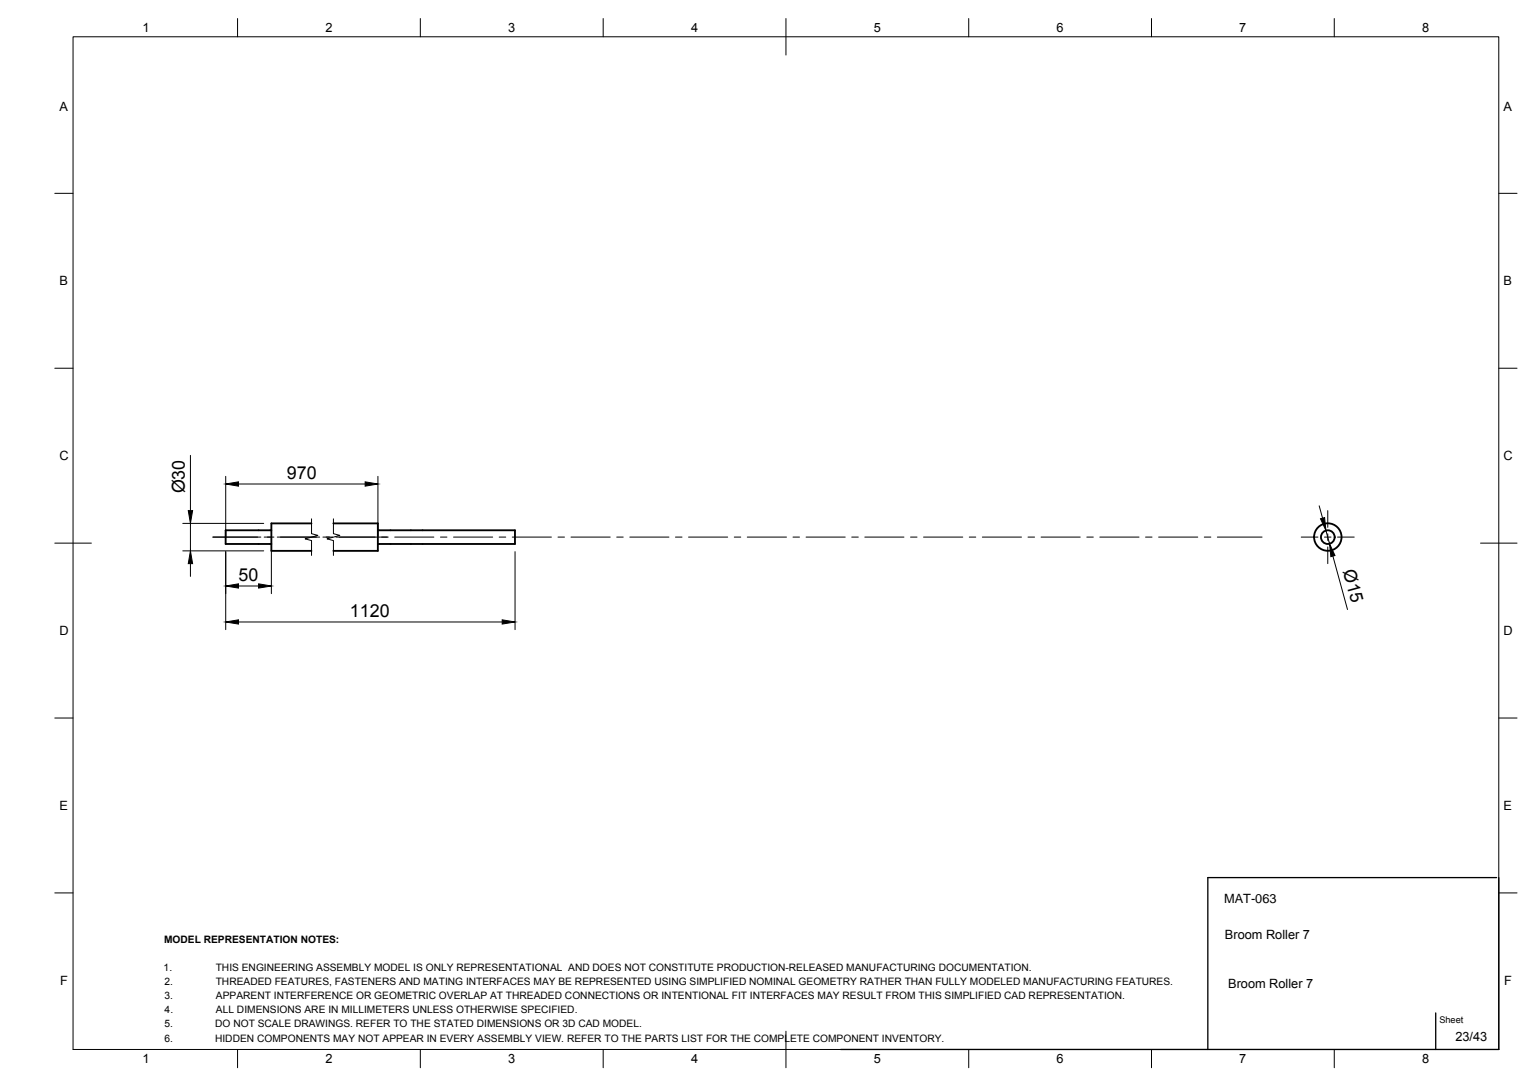
ISO-10303-21;
HEADER;
/* Generated by software containing ST-Developer
 * from STEP Tools, Inc. (www.steptools.com) 
 */

FILE_DESCRIPTION(
/* description */ (''),
/* implementation_level */ '2;1');

FILE_NAME(
/* name */ 'Broom Roller 7.step',
/* time_stamp */ '2026-10-24T09:43:01-07:00',
/* author */ (''),
/* organization */ (''),
/* preprocessor_version */ 'ST-DEVELOPER v20.2',
/* originating_system */ 'Autodesk Translation Framework v15.15.0.0',
/* authorisation */ '');

FILE_SCHEMA (('AUTOMOTIVE_DESIGN { 1 0 10303 214 3 1 1 }'));
ENDSEC;

DATA;
#10=MECHANICAL_DESIGN_GEOMETRIC_PRESENTATION_REPRESENTATION('',(#288),#11112);
#222=SHAPE_REPRESENTATION_RELATIONSHIP('SRR','None',#11246,#255);
#255=ADVANCED_BREP_SHAPE_REPRESENTATION('',(#321),#11091);
#288=STYLED_ITEM('',(#11426),#321);
#321=MANIFOLD_SOLID_BREP('Broom Roller 7',#6025);
#415=FACE_BOUND('',#1337,.T.);
#416=FACE_BOUND('',#1342,.T.);
#588=PLANE('',#6944);
#589=PLANE('',#6950);
#590=PLANE('',#6952);
#591=PLANE('',#6953);
#891=FACE_OUTER_BOUND('',#1331,.T.);
#892=FACE_OUTER_BOUND('',#1332,.T.);
#893=FACE_OUTER_BOUND('',#1333,.T.);
#894=FACE_OUTER_BOUND('',#1334,.T.);
#895=FACE_OUTER_BOUND('',#1335,.T.);
#896=FACE_OUTER_BOUND('',#1336,.T.);
#897=FACE_OUTER_BOUND('',#1338,.T.);
#898=FACE_OUTER_BOUND('',#1339,.T.);
#899=FACE_OUTER_BOUND('',#1340,.T.);
#900=FACE_OUTER_BOUND('',#1341,.T.);
#901=FACE_OUTER_BOUND('',#1343,.T.);
#902=FACE_OUTER_BOUND('',#1344,.T.);
#903=FACE_OUTER_BOUND('',#1345,.T.);
#1331=EDGE_LOOP('',(#4865,#4866,#4867,#4868,#4869,#4870));
#1332=EDGE_LOOP('',(#4871,#4872,#4873,#4874,#4875));
#1333=EDGE_LOOP('',(#4876,#4877,#4878,#4879,#4880));
#1334=EDGE_LOOP('',(#4881,#4882,#4883,#4884));
#1335=EDGE_LOOP('',(#4885,#4886,#4887,#4888));
#1336=EDGE_LOOP('',(#4889));
#1337=EDGE_LOOP('',(#4890));
#1338=EDGE_LOOP('',(#4891,#4892,#4893,#4894,#4895,#4896));
#1339=EDGE_LOOP('',(#4897,#4898,#4899,#4900));
#1340=EDGE_LOOP('',(#4901,#4902,#4903,#4904,#4905,#4906));
#1341=EDGE_LOOP('',(#4907));
#1342=EDGE_LOOP('',(#4908));
#1343=EDGE_LOOP('',(#4909,#4910,#4911,#4912));
#1344=EDGE_LOOP('',(#4913));
#1345=EDGE_LOOP('',(#4914));
#1732=LINE('',#10308,#2091);
#1733=LINE('',#10317,#2092);
#1734=LINE('',#10326,#2093);
#1735=LINE('',#10333,#2094);
#1736=LINE('',#10339,#2095);
#1737=LINE('',#10345,#2096);
#1738=LINE('',#10349,#2097);
#1739=LINE('',#10351,#2098);
#1740=LINE('',#10354,#2099);
#2091=VECTOR('',#8474,0.00749999975240883);
#2092=VECTOR('',#8485,0.00749999975240883);
#2093=VECTOR('',#8494,0.00749999975240883);
#2094=VECTOR('',#8503,0.00749999975240883);
#2095=VECTOR('',#8510,0.00749999975240883);
#2096=VECTOR('',#8519,0.0075);
#2097=VECTOR('',#8524,0.015);
#2098=VECTOR('',#8527,0.0075);
#2099=VECTOR('',#8532,0.0075);
#2558=CIRCLE('',#6926,0.00749999975240907);
#2559=CIRCLE('',#6927,0.0075);
#2560=CIRCLE('',#6928,0.0075);
#2561=CIRCLE('',#6929,0.00749999975240907);
#2562=CIRCLE('',#6931,0.00749999975240883);
#2563=CIRCLE('',#6932,0.0075);
#2564=CIRCLE('',#6933,0.0075);
#2565=CIRCLE('',#6935,0.00749999975240907);
#2566=CIRCLE('',#6936,0.00749999975240883);
#2567=CIRCLE('',#6937,0.00749999975240907);
#2568=CIRCLE('',#6939,0.0075);
#2569=CIRCLE('',#6940,0.00749999975240883);
#2570=CIRCLE('',#6942,0.00749999975240883);
#2571=CIRCLE('',#6943,0.00749999975240907);
#2572=CIRCLE('',#6945,0.015);
#2573=CIRCLE('',#6948,0.015);
#2968=VERTEX_POINT('',#10304);
#2969=VERTEX_POINT('',#10305);
#2970=VERTEX_POINT('',#10307);
#2971=VERTEX_POINT('',#10309);
#2972=VERTEX_POINT('',#10314);
#2973=VERTEX_POINT('',#10316);
#2974=VERTEX_POINT('',#10318);
#2975=VERTEX_POINT('',#10322);
#2976=VERTEX_POINT('',#10323);
#2977=VERTEX_POINT('',#10325);
#2978=VERTEX_POINT('',#10330);
#2979=VERTEX_POINT('',#10332);
#2980=VERTEX_POINT('',#10336);
#2981=VERTEX_POINT('',#10338);
#2982=VERTEX_POINT('',#10342);
#2983=VERTEX_POINT('',#10347);
#3636=EDGE_CURVE('',#2968,#2969,#2558,.T.);
#3637=EDGE_CURVE('',#2968,#2970,#1732,.T.);
#3638=EDGE_CURVE('',#2971,#2970,#2559,.F.);
#3639=EDGE_CURVE('',#2970,#2971,#2560,.F.);
#3640=EDGE_CURVE('',#2969,#2968,#2561,.T.);
#3641=EDGE_CURVE('',#2972,#2972,#2562,.T.);
#3642=EDGE_CURVE('',#2972,#2973,#1733,.T.);
#3643=EDGE_CURVE('',#2974,#2973,#2563,.F.);
#3644=EDGE_CURVE('',#2973,#2974,#2564,.F.);
#3645=EDGE_CURVE('',#2975,#2976,#2565,.T.);
#3646=EDGE_CURVE('',#2975,#2977,#1734,.T.);
#3647=EDGE_CURVE('',#2977,#2977,#2566,.T.);
#3648=EDGE_CURVE('',#2976,#2975,#2567,.T.);
#3649=EDGE_CURVE('',#2978,#2978,#2568,.F.);
#3650=EDGE_CURVE('',#2978,#2979,#1735,.T.);
#3651=EDGE_CURVE('',#2979,#2979,#2569,.T.);
#3652=EDGE_CURVE('',#2980,#2980,#2570,.T.);
#3653=EDGE_CURVE('',#2980,#2981,#1736,.T.);
#3654=EDGE_CURVE('',#2981,#2981,#2571,.T.);
#3655=EDGE_CURVE('',#2982,#2982,#2572,.T.);
#3656=EDGE_CURVE('',#2974,#2969,#1737,.T.);
#3657=EDGE_CURVE('',#2983,#2983,#2573,.T.);
#3658=EDGE_CURVE('',#2983,#2982,#1738,.T.);
#3659=EDGE_CURVE('',#2971,#2976,#1739,.T.);
#3660=EDGE_CURVE('',#2978,#2981,#1740,.T.);
#4865=ORIENTED_EDGE('',*,*,#3636,.F.);
#4866=ORIENTED_EDGE('',*,*,#3637,.T.);
#4867=ORIENTED_EDGE('',*,*,#3638,.F.);
#4868=ORIENTED_EDGE('',*,*,#3639,.F.);
#4869=ORIENTED_EDGE('',*,*,#3637,.F.);
#4870=ORIENTED_EDGE('',*,*,#3640,.F.);
#4871=ORIENTED_EDGE('',*,*,#3641,.F.);
#4872=ORIENTED_EDGE('',*,*,#3642,.T.);
#4873=ORIENTED_EDGE('',*,*,#3643,.F.);
#4874=ORIENTED_EDGE('',*,*,#3644,.F.);
#4875=ORIENTED_EDGE('',*,*,#3642,.F.);
#4876=ORIENTED_EDGE('',*,*,#3645,.F.);
#4877=ORIENTED_EDGE('',*,*,#3646,.T.);
#4878=ORIENTED_EDGE('',*,*,#3647,.F.);
#4879=ORIENTED_EDGE('',*,*,#3646,.F.);
#4880=ORIENTED_EDGE('',*,*,#3648,.F.);
#4881=ORIENTED_EDGE('',*,*,#3649,.F.);
#4882=ORIENTED_EDGE('',*,*,#3650,.T.);
#4883=ORIENTED_EDGE('',*,*,#3651,.F.);
#4884=ORIENTED_EDGE('',*,*,#3650,.F.);
#4885=ORIENTED_EDGE('',*,*,#3652,.F.);
#4886=ORIENTED_EDGE('',*,*,#3653,.T.);
#4887=ORIENTED_EDGE('',*,*,#3654,.F.);
#4888=ORIENTED_EDGE('',*,*,#3653,.F.);
#4889=ORIENTED_EDGE('',*,*,#3655,.F.);
#4890=ORIENTED_EDGE('',*,*,#3641,.T.);
#4891=ORIENTED_EDGE('',*,*,#3643,.T.);
#4892=ORIENTED_EDGE('',*,*,#3644,.T.);
#4893=ORIENTED_EDGE('',*,*,#3656,.T.);
#4894=ORIENTED_EDGE('',*,*,#3640,.T.);
#4895=ORIENTED_EDGE('',*,*,#3636,.T.);
#4896=ORIENTED_EDGE('',*,*,#3656,.F.);
#4897=ORIENTED_EDGE('',*,*,#3657,.T.);
#4898=ORIENTED_EDGE('',*,*,#3658,.T.);
#4899=ORIENTED_EDGE('',*,*,#3655,.T.);
#4900=ORIENTED_EDGE('',*,*,#3658,.F.);
#4901=ORIENTED_EDGE('',*,*,#3638,.T.);
#4902=ORIENTED_EDGE('',*,*,#3639,.T.);
#4903=ORIENTED_EDGE('',*,*,#3659,.T.);
#4904=ORIENTED_EDGE('',*,*,#3648,.T.);
#4905=ORIENTED_EDGE('',*,*,#3645,.T.);
#4906=ORIENTED_EDGE('',*,*,#3659,.F.);
#4907=ORIENTED_EDGE('',*,*,#3657,.F.);
#4908=ORIENTED_EDGE('',*,*,#3652,.T.);
#4909=ORIENTED_EDGE('',*,*,#3649,.T.);
#4910=ORIENTED_EDGE('',*,*,#3660,.T.);
#4911=ORIENTED_EDGE('',*,*,#3654,.T.);
#4912=ORIENTED_EDGE('',*,*,#3660,.F.);
#4913=ORIENTED_EDGE('',*,*,#3647,.T.);
#4914=ORIENTED_EDGE('',*,*,#3651,.T.);
#5577=CYLINDRICAL_SURFACE('',#6925,0.00749999975240883);
#5578=CYLINDRICAL_SURFACE('',#6930,0.00749999975240883);
#5579=CYLINDRICAL_SURFACE('',#6934,0.00749999975240883);
#5580=CYLINDRICAL_SURFACE('',#6938,0.00749999975240883);
#5581=CYLINDRICAL_SURFACE('',#6941,0.00749999975240883);
#5582=CYLINDRICAL_SURFACE('',#6946,0.0075);
#5583=CYLINDRICAL_SURFACE('',#6947,0.015);
#5584=CYLINDRICAL_SURFACE('',#6949,0.0075);
#5585=CYLINDRICAL_SURFACE('',#6951,0.0075);
#5864=ADVANCED_FACE('',(#891),#5577,.T.);
#5865=ADVANCED_FACE('',(#892),#5578,.T.);
#5866=ADVANCED_FACE('',(#893),#5579,.T.);
#5867=ADVANCED_FACE('',(#894),#5580,.T.);
#5868=ADVANCED_FACE('',(#895),#5581,.T.);
#5869=ADVANCED_FACE('',(#896,#415),#588,.F.);
#5870=ADVANCED_FACE('',(#897),#5582,.T.);
#5871=ADVANCED_FACE('',(#898),#5583,.T.);
#5872=ADVANCED_FACE('',(#899),#5584,.T.);
#5873=ADVANCED_FACE('',(#900,#416),#589,.F.);
#5874=ADVANCED_FACE('',(#901),#5585,.T.);
#5875=ADVANCED_FACE('',(#902),#590,.T.);
#5876=ADVANCED_FACE('',(#903),#591,.T.);
#6025=CLOSED_SHELL('',(#5864,#5865,#5866,#5867,#5868,#5869,#5870,#5871,
#5872,#5873,#5874,#5875,#5876));
#6924=AXIS2_PLACEMENT_3D('',#10302,#8468,#8469);
#6925=AXIS2_PLACEMENT_3D('',#10303,#8470,#8471);
#6926=AXIS2_PLACEMENT_3D('',#10306,#8472,#8473);
#6927=AXIS2_PLACEMENT_3D('',#10310,#8475,#8476);
#6928=AXIS2_PLACEMENT_3D('',#10311,#8477,#8478);
#6929=AXIS2_PLACEMENT_3D('',#10312,#8479,#8480);
#6930=AXIS2_PLACEMENT_3D('',#10313,#8481,#8482);
#6931=AXIS2_PLACEMENT_3D('',#10315,#8483,#8484);
#6932=AXIS2_PLACEMENT_3D('',#10319,#8486,#8487);
#6933=AXIS2_PLACEMENT_3D('',#10320,#8488,#8489);
#6934=AXIS2_PLACEMENT_3D('',#10321,#8490,#8491);
#6935=AXIS2_PLACEMENT_3D('',#10324,#8492,#8493);
#6936=AXIS2_PLACEMENT_3D('',#10327,#8495,#8496);
#6937=AXIS2_PLACEMENT_3D('',#10328,#8497,#8498);
#6938=AXIS2_PLACEMENT_3D('',#10329,#8499,#8500);
#6939=AXIS2_PLACEMENT_3D('',#10331,#8501,#8502);
#6940=AXIS2_PLACEMENT_3D('',#10334,#8504,#8505);
#6941=AXIS2_PLACEMENT_3D('',#10335,#8506,#8507);
#6942=AXIS2_PLACEMENT_3D('',#10337,#8508,#8509);
#6943=AXIS2_PLACEMENT_3D('',#10340,#8511,#8512);
#6944=AXIS2_PLACEMENT_3D('',#10341,#8513,#8514);
#6945=AXIS2_PLACEMENT_3D('',#10343,#8515,#8516);
#6946=AXIS2_PLACEMENT_3D('',#10344,#8517,#8518);
#6947=AXIS2_PLACEMENT_3D('',#10346,#8520,#8521);
#6948=AXIS2_PLACEMENT_3D('',#10348,#8522,#8523);
#6949=AXIS2_PLACEMENT_3D('',#10350,#8525,#8526);
#6950=AXIS2_PLACEMENT_3D('',#10352,#8528,#8529);
#6951=AXIS2_PLACEMENT_3D('',#10353,#8530,#8531);
#6952=AXIS2_PLACEMENT_3D('',#10355,#8533,#8534);
#6953=AXIS2_PLACEMENT_3D('',#10356,#8535,#8536);
#8468=DIRECTION('axis',(0.,0.,1.));
#8469=DIRECTION('refdir',(1.,0.,0.));
#8470=DIRECTION('center_axis',(-1.,0.,0.));
#8471=DIRECTION('ref_axis',(0.,0.464060113818661,0.885803708934779));
#8472=DIRECTION('center_axis',(1.,-1.0700065104041E-8,5.60561397559687E-9));
#8473=DIRECTION('ref_axis',(1.48029741503464E-16,-0.464060114221788,-0.885803708723587));
#8474=DIRECTION('',(-1.,0.,0.));
#8475=DIRECTION('center_axis',(1.,0.,0.));
#8476=DIRECTION('ref_axis',(0.,-0.464060130396268,-0.885803700250004));
#8477=DIRECTION('center_axis',(1.,0.,0.));
#8478=DIRECTION('ref_axis',(0.,-0.464060130396268,-0.885803700250004));
#8479=DIRECTION('center_axis',(1.,-1.0700065104041E-8,5.60561397559687E-9));
#8480=DIRECTION('ref_axis',(1.48029741503464E-16,-0.464060114221788,-0.885803708723587));
#8481=DIRECTION('center_axis',(-1.,0.,0.));
#8482=DIRECTION('ref_axis',(0.,0.464060113818661,0.885803708934779));
#8483=DIRECTION('center_axis',(1.,0.,0.));
#8484=DIRECTION('ref_axis',(0.,0.464060113818661,0.885803708934779));
#8485=DIRECTION('',(-1.,0.,0.));
#8486=DIRECTION('center_axis',(1.,0.,0.));
#8487=DIRECTION('ref_axis',(0.,-0.464060130396268,-0.885803700250004));
#8488=DIRECTION('center_axis',(1.,0.,0.));
#8489=DIRECTION('ref_axis',(0.,-0.464060130396268,-0.885803700250004));
#8490=DIRECTION('center_axis',(-1.,0.,0.));
#8491=DIRECTION('ref_axis',(0.,0.464060113818661,0.885803708934779));
#8492=DIRECTION('center_axis',(1.,-1.0700065104041E-8,5.60561397559687E-9));
#8493=DIRECTION('ref_axis',(1.48029741503464E-16,-0.464060114221788,-0.885803708723587));
#8494=DIRECTION('',(-1.,0.,0.));
#8495=DIRECTION('center_axis',(-1.,3.00553233246224E-15,2.27067042532096E-15));
#8496=DIRECTION('ref_axis',(0.,0.464060113818661,0.885803708934779));
#8497=DIRECTION('center_axis',(1.,-1.0700065104041E-8,5.60561397559687E-9));
#8498=DIRECTION('ref_axis',(1.48029741503464E-16,-0.464060114221788,-0.885803708723587));
#8499=DIRECTION('center_axis',(1.,0.,0.));
#8500=DIRECTION('ref_axis',(0.,-0.464060145800476,-0.885803692179955));
#8501=DIRECTION('center_axis',(1.,0.,0.));
#8502=DIRECTION('ref_axis',(0.,-0.464060130396268,-0.885803700250004));
#8503=DIRECTION('',(1.,0.,0.));
#8504=DIRECTION('center_axis',(1.,0.,0.));
#8505=DIRECTION('ref_axis',(0.,-0.464060145800476,-0.885803692179955));
#8506=DIRECTION('center_axis',(1.,0.,0.));
#8507=DIRECTION('ref_axis',(0.,-0.464060145800476,-0.885803692179955));
#8508=DIRECTION('center_axis',(-1.,0.,0.));
#8509=DIRECTION('ref_axis',(0.,-0.464060145800476,-0.885803692179955));
#8510=DIRECTION('',(1.,0.,0.));
#8511=DIRECTION('center_axis',(1.,-1.0700065104041E-8,5.60561397559687E-9));
#8512=DIRECTION('ref_axis',(1.48029741503464E-16,-0.464060114221788,-0.885803708723587));
#8513=DIRECTION('center_axis',(1.,8.31396011574228E-18,-4.70975743895875E-17));
#8514=DIRECTION('ref_axis',(-3.78610282642285E-17,-0.464060130015739,-0.885803700449358));
#8515=DIRECTION('center_axis',(1.,0.,0.));
#8516=DIRECTION('ref_axis',(0.,0.,-1.));
#8517=DIRECTION('center_axis',(1.,-5.36677334535434E-17,-1.02441631618442E-16));
#8518=DIRECTION('ref_axis',(-1.15648231731787E-16,-0.464060130015739,-0.885803700449358));
#8519=DIRECTION('',(-1.,5.36677334535434E-17,1.02441631618442E-16));
#8520=DIRECTION('center_axis',(1.,0.,0.));
#8521=DIRECTION('ref_axis',(0.,0.,-1.));
#8522=DIRECTION('center_axis',(-1.,0.,0.));
#8523=DIRECTION('ref_axis',(0.,0.,-1.));
#8524=DIRECTION('',(-1.,0.,0.));
#8525=DIRECTION('center_axis',(1.,-5.36677334535434E-17,-1.02441631618442E-16));
#8526=DIRECTION('ref_axis',(-1.15648231731787E-16,-0.464060130015739,-0.885803700449358));
#8527=DIRECTION('',(-1.,5.36677334535434E-17,1.02441631618442E-16));
#8528=DIRECTION('center_axis',(-1.,4.34535475133972E-17,1.99773034889551E-17));
#8529=DIRECTION('ref_axis',(3.78610282642285E-17,0.464060130015739,0.885803700449358));
#8530=DIRECTION('center_axis',(1.,-5.36677334535434E-17,-1.02441631618442E-16));
#8531=DIRECTION('ref_axis',(-1.15648231731787E-16,-0.464060130015739,-0.885803700449358));
#8532=DIRECTION('',(-1.,5.36677334535434E-17,1.02441631618442E-16));
#8533=DIRECTION('center_axis',(-1.,3.00553233246224E-15,2.27067042532096E-15));
#8534=DIRECTION('ref_axis',(-3.00553233246224E-15,-1.,4.51258949388147E-46));
#8535=DIRECTION('center_axis',(1.,0.,0.));
#8536=DIRECTION('ref_axis',(0.,0.,-1.));
#10302=CARTESIAN_POINT('',(0.,0.,0.));
#10303=CARTESIAN_POINT('Origin',(-0.459999999999996,0.350000000118451,1.09999999993794));
#10304=CARTESIAN_POINT('',(-0.473899999331871,0.346519549139845,1.09335647246591));
#10305=CARTESIAN_POINT('',(-0.473899999860731,0.353480450975115,1.10664352775337));
#10306=CARTESIAN_POINT('Origin',(-0.473899999770134,0.349999999881542,1.10000000006206));
#10307=CARTESIAN_POINT('',(-0.496099999999996,0.346519549379708,1.09335647234025));
#10308=CARTESIAN_POINT('',(-0.459999999999996,0.346519549379708,1.09335647234025));
#10309=CARTESIAN_POINT('',(-0.496100000552817,0.353480450914643,1.10664352764529));
#10310=CARTESIAN_POINT('Origin',(-0.496099999999996,0.349999999999997,1.1));
#10311=CARTESIAN_POINT('Origin',(-0.496099999999996,0.349999999999997,1.1));
#10312=CARTESIAN_POINT('Origin',(-0.473899999770134,0.349999999881542,1.10000000006206));
#10313=CARTESIAN_POINT('Origin',(-0.459999999999996,0.350000000118451,1.09999999993794));
#10314=CARTESIAN_POINT('',(-0.459999999999996,0.346519549379708,1.09335647234025));
#10315=CARTESIAN_POINT('Origin',(-0.459999999999996,0.350000000118451,1.09999999993794));
#10316=CARTESIAN_POINT('',(-0.461099999999996,0.346519549379708,1.09335647234025));
#10317=CARTESIAN_POINT('',(-0.459999999999996,0.346519549379708,1.09335647234025));
#10318=CARTESIAN_POINT('',(-0.461100000552817,0.353480450914643,1.10664352764529));
#10319=CARTESIAN_POINT('Origin',(-0.461099999999996,0.349999999999997,1.1));
#10320=CARTESIAN_POINT('Origin',(-0.461099999999996,0.349999999999997,1.1));
#10321=CARTESIAN_POINT('Origin',(-0.459999999999996,0.350000000118451,1.09999999993794));
#10322=CARTESIAN_POINT('',(-0.508899999331871,0.346519549139845,1.09335647246591));
#10323=CARTESIAN_POINT('',(-0.508899999860731,0.353480450975115,1.10664352775337));
#10324=CARTESIAN_POINT('Origin',(-0.508899999770134,0.349999999881542,1.10000000006206));
#10325=CARTESIAN_POINT('',(-0.61,0.346519549379708,1.09335647234025));
#10326=CARTESIAN_POINT('',(-0.459999999999996,0.346519549379708,1.09335647234025));
#10327=CARTESIAN_POINT('Origin',(-0.61,0.350000000118451,1.09999999993794));
#10328=CARTESIAN_POINT('Origin',(-0.508899999770134,0.349999999881542,1.10000000006206));
#10329=CARTESIAN_POINT('Origin',(0.46,0.350000000118451,1.09999999993794));
#10330=CARTESIAN_POINT('',(0.473899999447179,0.353480450914643,1.10664352764529));
#10331=CARTESIAN_POINT('Origin',(0.4739,0.349999999999997,1.1));
#10332=CARTESIAN_POINT('',(0.51,0.353480451097057,1.10664352740998));
#10333=CARTESIAN_POINT('',(0.46,0.353480451097057,1.10664352740998));
#10334=CARTESIAN_POINT('Origin',(0.51,0.350000000118451,1.09999999993794));
#10335=CARTESIAN_POINT('Origin',(0.46,0.350000000118451,1.09999999993794));
#10336=CARTESIAN_POINT('',(0.46,0.353480451097057,1.10664352740998));
#10337=CARTESIAN_POINT('Origin',(0.46,0.350000000118451,1.09999999993794));
#10338=CARTESIAN_POINT('',(0.461100000320458,0.353480451097057,1.10664352740998));
#10339=CARTESIAN_POINT('',(0.46,0.353480451097057,1.10664352740998));
#10340=CARTESIAN_POINT('Origin',(0.461100000229862,0.349999999881542,1.10000000006206));
#10341=CARTESIAN_POINT('Origin',(-0.459999999999996,0.349999999999997,1.1));
#10342=CARTESIAN_POINT('',(-0.459999999999996,0.35,1.115));
#10343=CARTESIAN_POINT('Origin',(-0.459999999999996,0.35,1.1));
#10344=CARTESIAN_POINT('Origin',(-0.488137499999996,0.349999999999997,1.1));
#10345=CARTESIAN_POINT('',(-0.488137499999996,0.353480450975115,1.10664352775337));
#10346=CARTESIAN_POINT('Origin',(-0.51,0.35,1.1));
#10347=CARTESIAN_POINT('',(0.46,0.35,1.115));
#10348=CARTESIAN_POINT('Origin',(0.46,0.35,1.1));
#10349=CARTESIAN_POINT('',(-0.51,0.35,1.115));
#10350=CARTESIAN_POINT('Origin',(-0.523137499999996,0.349999999999997,1.1));
#10351=CARTESIAN_POINT('',(-0.523137499999996,0.353480450975115,1.10664352775337));
#10352=CARTESIAN_POINT('Origin',(0.46,0.349999999999997,1.1));
#10353=CARTESIAN_POINT('Origin',(0.4468625,0.349999999999997,1.1));
#10354=CARTESIAN_POINT('',(0.4468625,0.353480450975115,1.10664352775337));
#10355=CARTESIAN_POINT('Origin',(-0.61,0.35,1.1));
#10356=CARTESIAN_POINT('Origin',(0.51,0.35,1.1));
#11052=UNCERTAINTY_MEASURE_WITH_UNIT(LENGTH_MEASURE(1.E-5),#11113,
'DISTANCE_ACCURACY_VALUE',
'Maximum model space distance between geometric entities at asserted c
onnectivities');
#11073=UNCERTAINTY_MEASURE_WITH_UNIT(LENGTH_MEASURE(1.E-5),#11113,
'DISTANCE_ACCURACY_VALUE',
'Maximum model space distance between geometric entities at asserted c
onnectivities');
#11091=(
GEOMETRIC_REPRESENTATION_CONTEXT(3)
GLOBAL_UNCERTAINTY_ASSIGNED_CONTEXT((#11052))
GLOBAL_UNIT_ASSIGNED_CONTEXT((#11113,#11114,#11115))
REPRESENTATION_CONTEXT('','3D')
);
#11112=(
GEOMETRIC_REPRESENTATION_CONTEXT(3)
GLOBAL_UNCERTAINTY_ASSIGNED_CONTEXT((#11073))
GLOBAL_UNIT_ASSIGNED_CONTEXT((#11113,#11114,#11115))
REPRESENTATION_CONTEXT('','3D')
);
#11113=(
LENGTH_UNIT()
NAMED_UNIT(*)
SI_UNIT($,.METRE.)
);
#11114=(
NAMED_UNIT(*)
PLANE_ANGLE_UNIT()
SI_UNIT($,.RADIAN.)
);
#11115=(
NAMED_UNIT(*)
SI_UNIT($,.STERADIAN.)
SOLID_ANGLE_UNIT()
);
#11133=SHAPE_DEFINITION_REPRESENTATION(#11171,#11246);
#11171=PRODUCT_DEFINITION_SHAPE('',$,#11285);
#11246=SHAPE_REPRESENTATION('',(#6924),#11091);
#11267=PRODUCT_DEFINITION_CONTEXT('part definition',#11383,'design');
#11285=PRODUCT_DEFINITION('Broom Roller 7','Broom Roller 7',#11323,#11267);
#11323=PRODUCT_DEFINITION_FORMATION('',$,#11402);
#11383=APPLICATION_CONTEXT(
'Core Data for Automotive Mechanical Design Process');
#11384=PRODUCT_CONTEXT('part definition',#11383,'mechanical');
#11402=PRODUCT('Broom Roller 7','Broom Roller 7',
'broom_and_roller__ DE     6017',(#11384));
#11426=PRESENTATION_STYLE_ASSIGNMENT((#11430));
#11430=SURFACE_STYLE_USAGE(.BOTH.,#11434);
#11434=SURFACE_SIDE_STYLE('',(#11438));
#11438=SURFACE_STYLE_FILL_AREA(#11442);
#11442=FILL_AREA_STYLE('Opaque(202,209,238)',(#11446));
#11446=FILL_AREA_STYLE_COLOUR('Opaque(202,209,238)',#11450);
#11450=COLOUR_RGB('Opaque(202,209,238)',0.792156862745098,0.819607843137255,
0.933333333333333);
ENDSEC;
END-ISO-10303-21;
